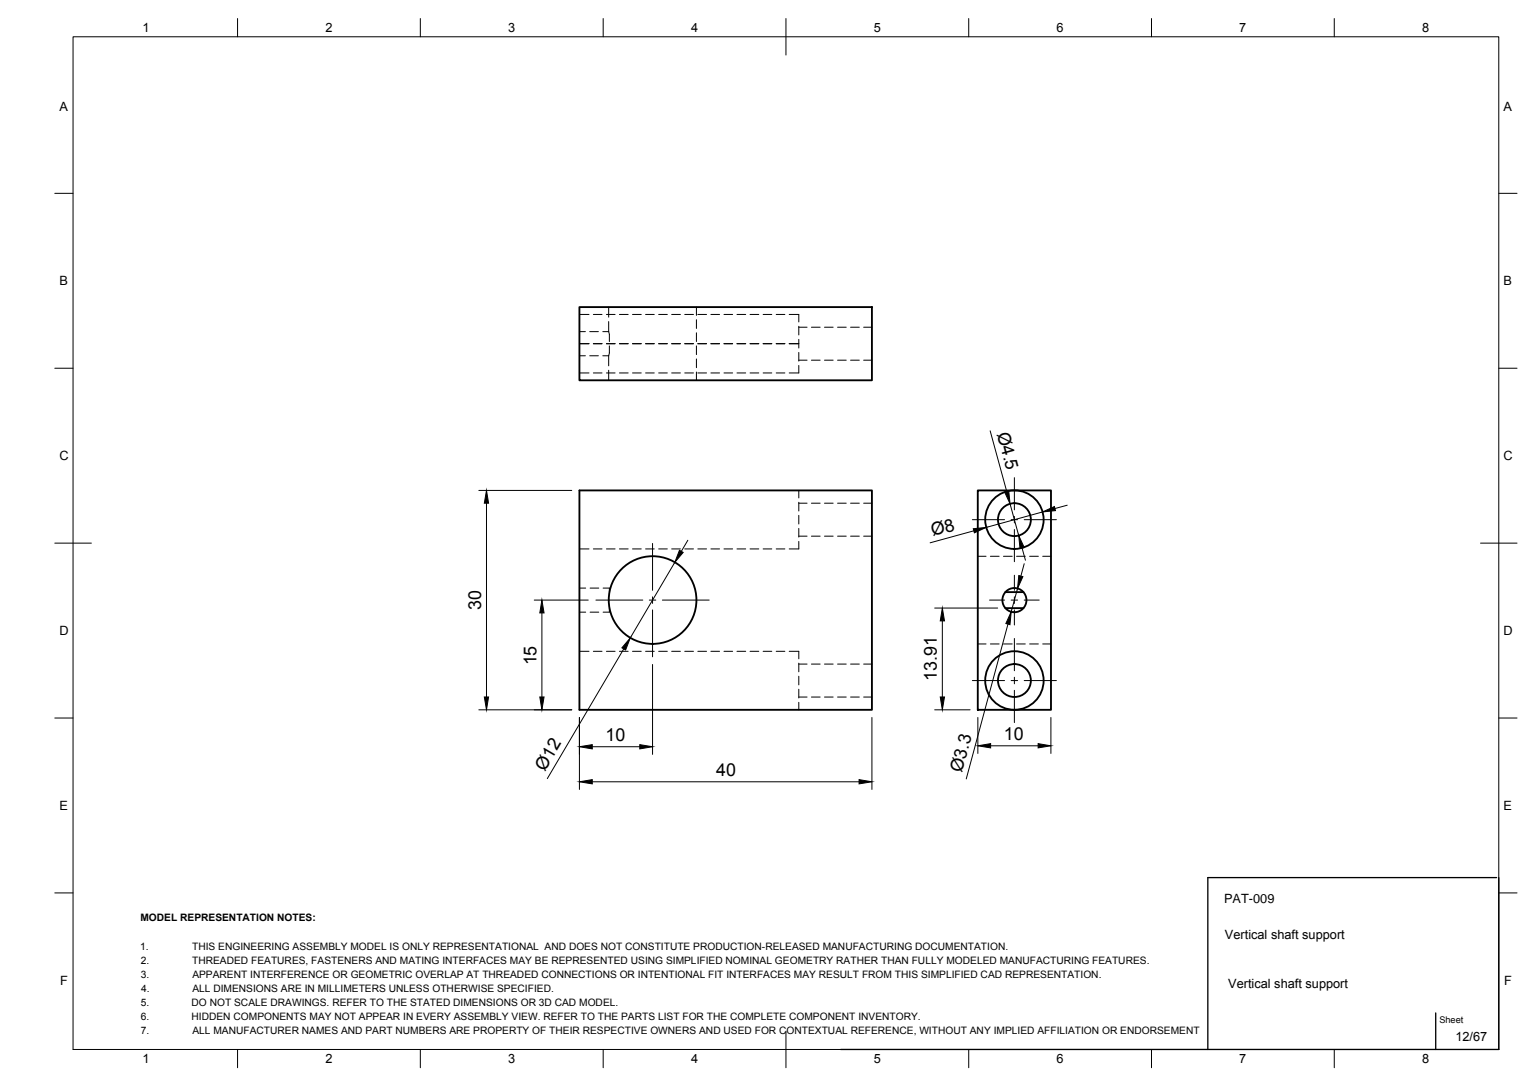
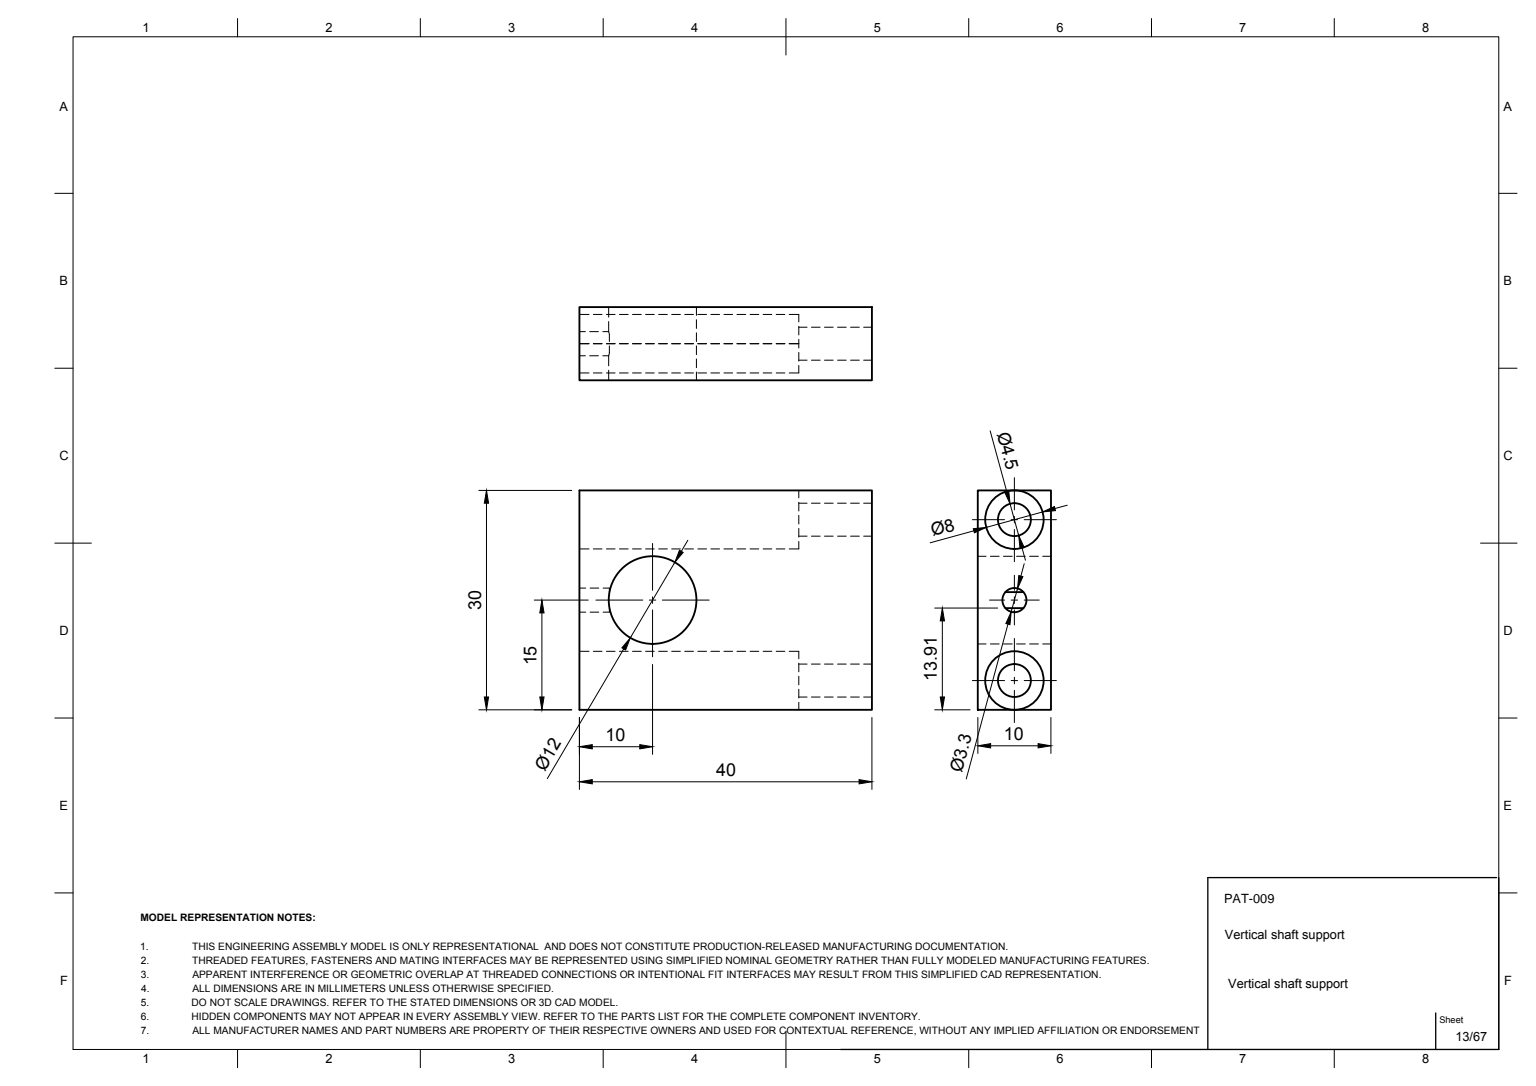
ISO-10303-21;
HEADER;
/* Generated by software containing ST-Developer
 * from STEP Tools, Inc. (www.steptools.com) 
 */

FILE_DESCRIPTION(
/* description */ ('Bell-crank linkage with push rods'),
/* implementation_level */ '2;1');

FILE_NAME(
/* name */ 'Vertical shaft support.step',
/* time_stamp */ '2026-10-28T03:25:15-07:00',
/* author */ (''),
/* organization */ (''),
/* preprocessor_version */ 'ST-DEVELOPER v20.2',
/* originating_system */ 'Autodesk Translation Framework v15.17.0.0',
/* authorisation */ '');

FILE_SCHEMA (('AUTOMOTIVE_DESIGN { 1 0 10303 214 3 1 1 }'));
ENDSEC;

DATA;
#10=MECHANICAL_DESIGN_GEOMETRIC_PRESENTATION_REPRESENTATION('',(#611),#16678);
#469=B_SPLINE_CURVE_WITH_KNOTS('',3,(#14216,#14217,#14218,#14219,#14220,
#14221,#14222,#14223,#14224,#14225),.UNSPECIFIED.,.F.,.F.,(4,2,2,2,4),(0.635430324955937,
0.687528937234029,0.750024497760675,0.81252005828732,0.864618670565412),
 .UNSPECIFIED.);
#470=B_SPLINE_CURVE_WITH_KNOTS('',3,(#14233,#14234,#14235,#14236,#14237,
#14238,#14239,#14240,#14241,#14242),.UNSPECIFIED.,.F.,.F.,(4,2,2,2,4),(0.135413993115487,
0.187512605393579,0.250008165920225,0.312503726446871,0.364602338724964),
 .UNSPECIFIED.);
#503=SHAPE_REPRESENTATION_RELATIONSHIP('SRR','None',#16919,#557);
#557=ADVANCED_BREP_SHAPE_REPRESENTATION('',(#673),#16624);
#611=STYLED_ITEM('',(#17291),#673);
#673=MANIFOLD_SOLID_BREP('Body1',#8801);
#796=FACE_BOUND('',#1959,.T.);
#797=FACE_BOUND('',#1962,.T.);
#798=FACE_BOUND('',#1964,.T.);
#799=FACE_BOUND('',#1968,.T.);
#800=FACE_BOUND('',#1970,.T.);
#801=FACE_BOUND('',#1973,.T.);
#802=FACE_BOUND('',#1976,.T.);
#803=FACE_BOUND('',#1977,.T.);
#1023=PLANE('',#9700);
#1024=PLANE('',#9706);
#1025=PLANE('',#9710);
#1026=PLANE('',#9715);
#1027=PLANE('',#9717);
#1028=PLANE('',#9725);
#1029=PLANE('',#9726);
#1030=PLANE('',#9727);
#1031=PLANE('',#9728);
#1032=PLANE('',#9729);
#1360=FACE_OUTER_BOUND('',#1953,.T.);
#1361=FACE_OUTER_BOUND('',#1954,.T.);
#1362=FACE_OUTER_BOUND('',#1955,.T.);
#1363=FACE_OUTER_BOUND('',#1956,.T.);
#1364=FACE_OUTER_BOUND('',#1957,.T.);
#1365=FACE_OUTER_BOUND('',#1958,.T.);
#1366=FACE_OUTER_BOUND('',#1960,.T.);
#1367=FACE_OUTER_BOUND('',#1961,.T.);
#1368=FACE_OUTER_BOUND('',#1963,.T.);
#1369=FACE_OUTER_BOUND('',#1965,.T.);
#1370=FACE_OUTER_BOUND('',#1966,.T.);
#1371=FACE_OUTER_BOUND('',#1967,.T.);
#1372=FACE_OUTER_BOUND('',#1969,.T.);
#1373=FACE_OUTER_BOUND('',#1971,.T.);
#1374=FACE_OUTER_BOUND('',#1972,.T.);
#1375=FACE_OUTER_BOUND('',#1974,.T.);
#1376=FACE_OUTER_BOUND('',#1975,.T.);
#1953=EDGE_LOOP('',(#6443,#6444,#6445,#6446));
#1954=EDGE_LOOP('',(#6447,#6448));
#1955=EDGE_LOOP('',(#6449,#6450,#6451,#6452,#6453,#6454,#6455,#6456));
#1956=EDGE_LOOP('',(#6457,#6458,#6459));
#1957=EDGE_LOOP('',(#6460,#6461,#6462,#6463));
#1958=EDGE_LOOP('',(#6464));
#1959=EDGE_LOOP('',(#6465));
#1960=EDGE_LOOP('',(#6466,#6467,#6468,#6469));
#1961=EDGE_LOOP('',(#6470,#6471));
#1962=EDGE_LOOP('',(#6472));
#1963=EDGE_LOOP('',(#6473,#6474,#6475,#6476,#6477,#6478,#6479,#6480,#6481));
#1964=EDGE_LOOP('',(#6482));
#1965=EDGE_LOOP('',(#6483,#6484,#6485,#6486));
#1966=EDGE_LOOP('',(#6487,#6488,#6489,#6490));
#1967=EDGE_LOOP('',(#6491,#6492,#6493,#6494));
#1968=EDGE_LOOP('',(#6495,#6496,#6497,#6498));
#1969=EDGE_LOOP('',(#6499,#6500,#6501,#6502));
#1970=EDGE_LOOP('',(#6503));
#1971=EDGE_LOOP('',(#6504,#6505,#6506,#6507,#6508,#6509,#6510));
#1972=EDGE_LOOP('',(#6511,#6512,#6513,#6514));
#1973=EDGE_LOOP('',(#6515));
#1974=EDGE_LOOP('',(#6516,#6517,#6518,#6519,#6520,#6521,#6522));
#1975=EDGE_LOOP('',(#6523,#6524,#6525,#6526));
#1976=EDGE_LOOP('',(#6527));
#1977=EDGE_LOOP('',(#6528));
#2666=LINE('',#14203,#3215);
#2667=LINE('',#14207,#3216);
#2668=LINE('',#14212,#3217);
#2669=LINE('',#14229,#3218);
#2670=LINE('',#14244,#3219);
#2671=LINE('',#14249,#3220);
#2672=LINE('',#14251,#3221);
#2673=LINE('',#14257,#3222);
#2674=LINE('',#14264,#3223);
#2675=LINE('',#14266,#3224);
#2676=LINE('',#14268,#3225);
#2677=LINE('',#14269,#3226);
#2678=LINE('',#14271,#3227);
#2679=LINE('',#14272,#3228);
#2680=LINE('',#14276,#3229);
#2681=LINE('',#14280,#3230);
#2682=LINE('',#14285,#3231);
#2683=LINE('',#14290,#3232);
#2684=LINE('',#14291,#3233);
#2685=LINE('',#14292,#3234);
#2686=LINE('',#14295,#3235);
#2687=LINE('',#14296,#3236);
#2688=LINE('',#14299,#3237);
#2689=LINE('',#14300,#3238);
#2690=LINE('',#14302,#3239);
#3215=VECTOR('',#11252,0.4);
#3216=VECTOR('',#11255,1.);
#3217=VECTOR('',#11260,1.);
#3218=VECTOR('',#11267,0.165);
#3219=VECTOR('',#11274,1.);
#3220=VECTOR('',#11279,1.);
#3221=VECTOR('',#11282,1.);
#3222=VECTOR('',#11291,1.);
#3223=VECTOR('',#11300,1.);
#3224=VECTOR('',#11301,1.);
#3225=VECTOR('',#11302,1.);
#3226=VECTOR('',#11303,1.);
#3227=VECTOR('',#11304,1.);
#3228=VECTOR('',#11305,1.);
#3229=VECTOR('',#11310,0.225);
#3230=VECTOR('',#11315,0.225);
#3231=VECTOR('',#11320,0.6);
#3232=VECTOR('',#11325,1.);
#3233=VECTOR('',#11326,1.);
#3234=VECTOR('',#11327,1.);
#3235=VECTOR('',#11330,1.);
#3236=VECTOR('',#11331,1.);
#3237=VECTOR('',#11334,1.);
#3238=VECTOR('',#11335,1.);
#3239=VECTOR('',#11338,1.);
#3750=CIRCLE('',#9698,0.4);
#3751=CIRCLE('',#9699,0.4);
#3752=CIRCLE('',#9701,0.165);
#3753=CIRCLE('',#9703,0.165);
#3754=CIRCLE('',#9704,0.165);
#3755=CIRCLE('',#9705,0.165);
#3756=CIRCLE('',#9708,0.4);
#3757=CIRCLE('',#9709,0.4);
#3758=CIRCLE('',#9711,0.225);
#3759=CIRCLE('',#9713,0.4);
#3760=CIRCLE('',#9714,0.4);
#3761=CIRCLE('',#9716,0.225);
#3762=CIRCLE('',#9719,0.225);
#3763=CIRCLE('',#9721,0.225);
#3764=CIRCLE('',#9723,0.6);
#3765=CIRCLE('',#9724,0.6);
#4292=VERTEX_POINT('',#14201);
#4293=VERTEX_POINT('',#14202);
#4294=VERTEX_POINT('',#14204);
#4295=VERTEX_POINT('',#14206);
#4296=VERTEX_POINT('',#14210);
#4297=VERTEX_POINT('',#14211);
#4298=VERTEX_POINT('',#14215);
#4299=VERTEX_POINT('',#14226);
#4300=VERTEX_POINT('',#14228);
#4301=VERTEX_POINT('',#14231);
#4302=VERTEX_POINT('',#14246);
#4303=VERTEX_POINT('',#14248);
#4304=VERTEX_POINT('',#14253);
#4305=VERTEX_POINT('',#14260);
#4306=VERTEX_POINT('',#14263);
#4307=VERTEX_POINT('',#14265);
#4308=VERTEX_POINT('',#14267);
#4309=VERTEX_POINT('',#14270);
#4310=VERTEX_POINT('',#14274);
#4311=VERTEX_POINT('',#14278);
#4312=VERTEX_POINT('',#14282);
#4313=VERTEX_POINT('',#14284);
#4314=VERTEX_POINT('',#14288);
#4315=VERTEX_POINT('',#14289);
#4316=VERTEX_POINT('',#14294);
#4317=VERTEX_POINT('',#14298);
#5099=EDGE_CURVE('',#4292,#4293,#2666,.T.);
#5100=EDGE_CURVE('',#4294,#4292,#3750,.T.);
#5101=EDGE_CURVE('',#4294,#4295,#2667,.T.);
#5102=EDGE_CURVE('',#4293,#4295,#3751,.T.);
#5103=EDGE_CURVE('',#4296,#4297,#2668,.T.);
#5104=EDGE_CURVE('',#4296,#4297,#3752,.T.);
#5105=EDGE_CURVE('',#4298,#4296,#469,.T.);
#5106=EDGE_CURVE('',#4299,#4298,#3753,.T.);
#5107=EDGE_CURVE('',#4299,#4300,#2669,.T.);
#5108=EDGE_CURVE('',#4300,#4300,#3754,.T.);
#5109=EDGE_CURVE('',#4301,#4299,#3755,.T.);
#5110=EDGE_CURVE('',#4297,#4301,#470,.T.);
#5111=EDGE_CURVE('',#4301,#4298,#2670,.T.);
#5112=EDGE_CURVE('',#4302,#4302,#3756,.T.);
#5113=EDGE_CURVE('',#4302,#4303,#2671,.T.);
#5114=EDGE_CURVE('',#4303,#4303,#3757,.T.);
#5115=EDGE_CURVE('',#4302,#4303,#2672,.T.);
#5116=EDGE_CURVE('',#4304,#4304,#3758,.T.);
#5117=EDGE_CURVE('',#4295,#4293,#3759,.T.);
#5118=EDGE_CURVE('',#4294,#4295,#2673,.T.);
#5119=EDGE_CURVE('',#4292,#4294,#3760,.T.);
#5120=EDGE_CURVE('',#4305,#4305,#3761,.T.);
#5121=EDGE_CURVE('',#4306,#4303,#2674,.T.);
#5122=EDGE_CURVE('',#4303,#4307,#2675,.T.);
#5123=EDGE_CURVE('',#4307,#4308,#2676,.T.);
#5124=EDGE_CURVE('',#4308,#4295,#2677,.T.);
#5125=EDGE_CURVE('',#4295,#4309,#2678,.T.);
#5126=EDGE_CURVE('',#4309,#4306,#2679,.T.);
#5127=EDGE_CURVE('',#4310,#4310,#3762,.T.);
#5128=EDGE_CURVE('',#4310,#4304,#2680,.T.);
#5129=EDGE_CURVE('',#4311,#4311,#3763,.T.);
#5130=EDGE_CURVE('',#4311,#4305,#2681,.T.);
#5131=EDGE_CURVE('',#4312,#4312,#3764,.T.);
#5132=EDGE_CURVE('',#4312,#4313,#2682,.T.);
#5133=EDGE_CURVE('',#4313,#4313,#3765,.T.);
#5134=EDGE_CURVE('',#4314,#4315,#2683,.T.);
#5135=EDGE_CURVE('',#4315,#4306,#2684,.T.);
#5136=EDGE_CURVE('',#4314,#4309,#2685,.T.);
#5137=EDGE_CURVE('',#4316,#4314,#2686,.T.);
#5138=EDGE_CURVE('',#4316,#4308,#2687,.T.);
#5139=EDGE_CURVE('',#4317,#4316,#2688,.T.);
#5140=EDGE_CURVE('',#4317,#4307,#2689,.T.);
#5141=EDGE_CURVE('',#4315,#4317,#2690,.T.);
#6443=ORIENTED_EDGE('',*,*,#5099,.F.);
#6444=ORIENTED_EDGE('',*,*,#5100,.F.);
#6445=ORIENTED_EDGE('',*,*,#5101,.T.);
#6446=ORIENTED_EDGE('',*,*,#5102,.F.);
#6447=ORIENTED_EDGE('',*,*,#5103,.F.);
#6448=ORIENTED_EDGE('',*,*,#5104,.T.);
#6449=ORIENTED_EDGE('',*,*,#5105,.F.);
#6450=ORIENTED_EDGE('',*,*,#5106,.F.);
#6451=ORIENTED_EDGE('',*,*,#5107,.T.);
#6452=ORIENTED_EDGE('',*,*,#5108,.F.);
#6453=ORIENTED_EDGE('',*,*,#5107,.F.);
#6454=ORIENTED_EDGE('',*,*,#5109,.F.);
#6455=ORIENTED_EDGE('',*,*,#5110,.F.);
#6456=ORIENTED_EDGE('',*,*,#5104,.F.);
#6457=ORIENTED_EDGE('',*,*,#5111,.F.);
#6458=ORIENTED_EDGE('',*,*,#5109,.T.);
#6459=ORIENTED_EDGE('',*,*,#5106,.T.);
#6460=ORIENTED_EDGE('',*,*,#5112,.F.);
#6461=ORIENTED_EDGE('',*,*,#5113,.T.);
#6462=ORIENTED_EDGE('',*,*,#5114,.F.);
#6463=ORIENTED_EDGE('',*,*,#5115,.F.);
#6464=ORIENTED_EDGE('',*,*,#5112,.T.);
#6465=ORIENTED_EDGE('',*,*,#5116,.F.);
#6466=ORIENTED_EDGE('',*,*,#5099,.T.);
#6467=ORIENTED_EDGE('',*,*,#5117,.F.);
#6468=ORIENTED_EDGE('',*,*,#5118,.F.);
#6469=ORIENTED_EDGE('',*,*,#5119,.F.);
#6470=ORIENTED_EDGE('',*,*,#5100,.T.);
#6471=ORIENTED_EDGE('',*,*,#5119,.T.);
#6472=ORIENTED_EDGE('',*,*,#5120,.F.);
#6473=ORIENTED_EDGE('',*,*,#5121,.T.);
#6474=ORIENTED_EDGE('',*,*,#5114,.T.);
#6475=ORIENTED_EDGE('',*,*,#5122,.T.);
#6476=ORIENTED_EDGE('',*,*,#5123,.T.);
#6477=ORIENTED_EDGE('',*,*,#5124,.T.);
#6478=ORIENTED_EDGE('',*,*,#5117,.T.);
#6479=ORIENTED_EDGE('',*,*,#5102,.T.);
#6480=ORIENTED_EDGE('',*,*,#5125,.T.);
#6481=ORIENTED_EDGE('',*,*,#5126,.T.);
#6482=ORIENTED_EDGE('',*,*,#5108,.T.);
#6483=ORIENTED_EDGE('',*,*,#5127,.F.);
#6484=ORIENTED_EDGE('',*,*,#5128,.T.);
#6485=ORIENTED_EDGE('',*,*,#5116,.T.);
#6486=ORIENTED_EDGE('',*,*,#5128,.F.);
#6487=ORIENTED_EDGE('',*,*,#5129,.F.);
#6488=ORIENTED_EDGE('',*,*,#5130,.T.);
#6489=ORIENTED_EDGE('',*,*,#5120,.T.);
#6490=ORIENTED_EDGE('',*,*,#5130,.F.);
#6491=ORIENTED_EDGE('',*,*,#5131,.F.);
#6492=ORIENTED_EDGE('',*,*,#5132,.T.);
#6493=ORIENTED_EDGE('',*,*,#5133,.F.);
#6494=ORIENTED_EDGE('',*,*,#5132,.F.);
#6495=ORIENTED_EDGE('',*,*,#5110,.T.);
#6496=ORIENTED_EDGE('',*,*,#5111,.T.);
#6497=ORIENTED_EDGE('',*,*,#5105,.T.);
#6498=ORIENTED_EDGE('',*,*,#5103,.T.);
#6499=ORIENTED_EDGE('',*,*,#5134,.T.);
#6500=ORIENTED_EDGE('',*,*,#5135,.T.);
#6501=ORIENTED_EDGE('',*,*,#5126,.F.);
#6502=ORIENTED_EDGE('',*,*,#5136,.F.);
#6503=ORIENTED_EDGE('',*,*,#5133,.T.);
#6504=ORIENTED_EDGE('',*,*,#5137,.T.);
#6505=ORIENTED_EDGE('',*,*,#5136,.T.);
#6506=ORIENTED_EDGE('',*,*,#5125,.F.);
#6507=ORIENTED_EDGE('',*,*,#5101,.F.);
#6508=ORIENTED_EDGE('',*,*,#5118,.T.);
#6509=ORIENTED_EDGE('',*,*,#5124,.F.);
#6510=ORIENTED_EDGE('',*,*,#5138,.F.);
#6511=ORIENTED_EDGE('',*,*,#5139,.T.);
#6512=ORIENTED_EDGE('',*,*,#5138,.T.);
#6513=ORIENTED_EDGE('',*,*,#5123,.F.);
#6514=ORIENTED_EDGE('',*,*,#5140,.F.);
#6515=ORIENTED_EDGE('',*,*,#5131,.T.);
#6516=ORIENTED_EDGE('',*,*,#5141,.T.);
#6517=ORIENTED_EDGE('',*,*,#5140,.T.);
#6518=ORIENTED_EDGE('',*,*,#5122,.F.);
#6519=ORIENTED_EDGE('',*,*,#5113,.F.);
#6520=ORIENTED_EDGE('',*,*,#5115,.T.);
#6521=ORIENTED_EDGE('',*,*,#5121,.F.);
#6522=ORIENTED_EDGE('',*,*,#5135,.F.);
#6523=ORIENTED_EDGE('',*,*,#5141,.F.);
#6524=ORIENTED_EDGE('',*,*,#5134,.F.);
#6525=ORIENTED_EDGE('',*,*,#5137,.F.);
#6526=ORIENTED_EDGE('',*,*,#5139,.F.);
#6527=ORIENTED_EDGE('',*,*,#5127,.T.);
#6528=ORIENTED_EDGE('',*,*,#5129,.T.);
#8123=CYLINDRICAL_SURFACE('',#9697,0.4);
#8124=CYLINDRICAL_SURFACE('',#9702,0.165);
#8125=CYLINDRICAL_SURFACE('',#9707,0.4);
#8126=CYLINDRICAL_SURFACE('',#9712,0.4);
#8127=CYLINDRICAL_SURFACE('',#9718,0.225);
#8128=CYLINDRICAL_SURFACE('',#9720,0.225);
#8129=CYLINDRICAL_SURFACE('',#9722,0.6);
#8385=ADVANCED_FACE('',(#1360),#8123,.F.);
#8386=ADVANCED_FACE('',(#1361),#1023,.T.);
#8387=ADVANCED_FACE('',(#1362),#8124,.F.);
#8388=ADVANCED_FACE('',(#1363),#1024,.T.);
#8389=ADVANCED_FACE('',(#1364),#8125,.F.);
#8390=ADVANCED_FACE('',(#1365,#796),#1025,.T.);
#8391=ADVANCED_FACE('',(#1366),#8126,.F.);
#8392=ADVANCED_FACE('',(#1367,#797),#1026,.T.);
#8393=ADVANCED_FACE('',(#1368,#798),#1027,.T.);
#8394=ADVANCED_FACE('',(#1369),#8127,.F.);
#8395=ADVANCED_FACE('',(#1370),#8128,.F.);
#8396=ADVANCED_FACE('',(#1371,#799),#8129,.F.);
#8397=ADVANCED_FACE('',(#1372,#800),#1028,.T.);
#8398=ADVANCED_FACE('',(#1373),#1029,.T.);
#8399=ADVANCED_FACE('',(#1374,#801),#1030,.T.);
#8400=ADVANCED_FACE('',(#1375),#1031,.T.);
#8401=ADVANCED_FACE('',(#1376,#802,#803),#1032,.F.);
#8801=CLOSED_SHELL('',(#8385,#8386,#8387,#8388,#8389,#8390,#8391,#8392,
#8393,#8394,#8395,#8396,#8397,#8398,#8399,#8400,#8401));
#9696=AXIS2_PLACEMENT_3D('',#14199,#11248,#11249);
#9697=AXIS2_PLACEMENT_3D('',#14200,#11250,#11251);
#9698=AXIS2_PLACEMENT_3D('',#14205,#11253,#11254);
#9699=AXIS2_PLACEMENT_3D('',#14208,#11256,#11257);
#9700=AXIS2_PLACEMENT_3D('',#14209,#11258,#11259);
#9701=AXIS2_PLACEMENT_3D('',#14213,#11261,#11262);
#9702=AXIS2_PLACEMENT_3D('',#14214,#11263,#11264);
#9703=AXIS2_PLACEMENT_3D('',#14227,#11265,#11266);
#9704=AXIS2_PLACEMENT_3D('',#14230,#11268,#11269);
#9705=AXIS2_PLACEMENT_3D('',#14232,#11270,#11271);
#9706=AXIS2_PLACEMENT_3D('',#14243,#11272,#11273);
#9707=AXIS2_PLACEMENT_3D('',#14245,#11275,#11276);
#9708=AXIS2_PLACEMENT_3D('',#14247,#11277,#11278);
#9709=AXIS2_PLACEMENT_3D('',#14250,#11280,#11281);
#9710=AXIS2_PLACEMENT_3D('',#14252,#11283,#11284);
#9711=AXIS2_PLACEMENT_3D('',#14254,#11285,#11286);
#9712=AXIS2_PLACEMENT_3D('',#14255,#11287,#11288);
#9713=AXIS2_PLACEMENT_3D('',#14256,#11289,#11290);
#9714=AXIS2_PLACEMENT_3D('',#14258,#11292,#11293);
#9715=AXIS2_PLACEMENT_3D('',#14259,#11294,#11295);
#9716=AXIS2_PLACEMENT_3D('',#14261,#11296,#11297);
#9717=AXIS2_PLACEMENT_3D('',#14262,#11298,#11299);
#9718=AXIS2_PLACEMENT_3D('',#14273,#11306,#11307);
#9719=AXIS2_PLACEMENT_3D('',#14275,#11308,#11309);
#9720=AXIS2_PLACEMENT_3D('',#14277,#11311,#11312);
#9721=AXIS2_PLACEMENT_3D('',#14279,#11313,#11314);
#9722=AXIS2_PLACEMENT_3D('',#14281,#11316,#11317);
#9723=AXIS2_PLACEMENT_3D('',#14283,#11318,#11319);
#9724=AXIS2_PLACEMENT_3D('',#14286,#11321,#11322);
#9725=AXIS2_PLACEMENT_3D('',#14287,#11323,#11324);
#9726=AXIS2_PLACEMENT_3D('',#14293,#11328,#11329);
#9727=AXIS2_PLACEMENT_3D('',#14297,#11332,#11333);
#9728=AXIS2_PLACEMENT_3D('',#14301,#11336,#11337);
#9729=AXIS2_PLACEMENT_3D('',#14303,#11339,#11340);
#11248=DIRECTION('axis',(0.,0.,1.));
#11249=DIRECTION('refdir',(1.,0.,0.));
#11250=DIRECTION('center_axis',(0.,0.,1.));
#11251=DIRECTION('ref_axis',(1.,0.,0.));
#11252=DIRECTION('',(0.,0.,1.));
#11253=DIRECTION('center_axis',(0.,0.,1.));
#11254=DIRECTION('ref_axis',(1.,0.,0.));
#11255=DIRECTION('',(0.,0.,1.));
#11256=DIRECTION('center_axis',(0.,0.,-1.));
#11257=DIRECTION('ref_axis',(1.,0.,0.));
#11258=DIRECTION('center_axis',(0.,0.,1.));
#11259=DIRECTION('ref_axis',(1.,0.,0.));
#11260=DIRECTION('',(0.,1.,0.));
#11261=DIRECTION('center_axis',(0.,0.,1.));
#11262=DIRECTION('ref_axis',(1.,0.,0.));
#11263=DIRECTION('center_axis',(0.,0.,1.));
#11264=DIRECTION('ref_axis',(1.,0.,0.));
#11265=DIRECTION('center_axis',(0.,0.,1.));
#11266=DIRECTION('ref_axis',(1.,0.,0.));
#11267=DIRECTION('',(0.,0.,1.));
#11268=DIRECTION('center_axis',(0.,0.,-1.));
#11269=DIRECTION('ref_axis',(1.,0.,0.));
#11270=DIRECTION('center_axis',(0.,0.,1.));
#11271=DIRECTION('ref_axis',(1.,0.,0.));
#11272=DIRECTION('center_axis',(0.,0.,1.));
#11273=DIRECTION('ref_axis',(1.,0.,0.));
#11274=DIRECTION('',(0.,-1.,0.));
#11275=DIRECTION('center_axis',(0.,0.,1.));
#11276=DIRECTION('ref_axis',(1.,0.,0.));
#11277=DIRECTION('center_axis',(0.,0.,1.));
#11278=DIRECTION('ref_axis',(1.,0.,0.));
#11279=DIRECTION('',(0.,0.,1.));
#11280=DIRECTION('center_axis',(0.,0.,-1.));
#11281=DIRECTION('ref_axis',(1.,0.,0.));
#11282=DIRECTION('',(0.,0.,1.));
#11283=DIRECTION('center_axis',(0.,0.,1.));
#11284=DIRECTION('ref_axis',(1.,0.,0.));
#11285=DIRECTION('center_axis',(0.,0.,1.));
#11286=DIRECTION('ref_axis',(1.,0.,0.));
#11287=DIRECTION('center_axis',(0.,0.,1.));
#11288=DIRECTION('ref_axis',(1.,0.,0.));
#11289=DIRECTION('center_axis',(0.,0.,-1.));
#11290=DIRECTION('ref_axis',(1.,0.,0.));
#11291=DIRECTION('',(0.,0.,1.));
#11292=DIRECTION('center_axis',(0.,0.,1.));
#11293=DIRECTION('ref_axis',(1.,0.,0.));
#11294=DIRECTION('center_axis',(0.,0.,1.));
#11295=DIRECTION('ref_axis',(1.,0.,0.));
#11296=DIRECTION('center_axis',(0.,0.,1.));
#11297=DIRECTION('ref_axis',(1.,0.,0.));
#11298=DIRECTION('center_axis',(0.,0.,1.));
#11299=DIRECTION('ref_axis',(1.,0.,0.));
#11300=DIRECTION('',(0.,-1.,0.));
#11301=DIRECTION('',(0.,-1.,0.));
#11302=DIRECTION('',(1.,0.,0.));
#11303=DIRECTION('',(0.,1.,0.));
#11304=DIRECTION('',(0.,1.,0.));
#11305=DIRECTION('',(-1.,0.,0.));
#11306=DIRECTION('center_axis',(0.,0.,1.));
#11307=DIRECTION('ref_axis',(1.,0.,0.));
#11308=DIRECTION('center_axis',(0.,0.,1.));
#11309=DIRECTION('ref_axis',(1.,0.,0.));
#11310=DIRECTION('',(0.,0.,1.));
#11311=DIRECTION('center_axis',(0.,0.,1.));
#11312=DIRECTION('ref_axis',(1.,0.,0.));
#11313=DIRECTION('center_axis',(0.,0.,1.));
#11314=DIRECTION('ref_axis',(1.,0.,0.));
#11315=DIRECTION('',(0.,0.,1.));
#11316=DIRECTION('center_axis',(0.,1.,0.));
#11317=DIRECTION('ref_axis',(1.,0.,0.));
#11318=DIRECTION('center_axis',(0.,1.,0.));
#11319=DIRECTION('ref_axis',(1.,0.,0.));
#11320=DIRECTION('',(0.,1.,0.));
#11321=DIRECTION('center_axis',(0.,-1.,0.));
#11322=DIRECTION('ref_axis',(1.,0.,0.));
#11323=DIRECTION('center_axis',(0.,1.,0.));
#11324=DIRECTION('ref_axis',(-1.,0.,0.));
#11325=DIRECTION('',(-1.,0.,0.));
#11326=DIRECTION('',(0.,0.,1.));
#11327=DIRECTION('',(0.,0.,1.));
#11328=DIRECTION('center_axis',(1.,0.,0.));
#11329=DIRECTION('ref_axis',(0.,1.,0.));
#11330=DIRECTION('',(0.,1.,0.));
#11331=DIRECTION('',(0.,0.,1.));
#11332=DIRECTION('center_axis',(0.,-1.,0.));
#11333=DIRECTION('ref_axis',(1.,0.,0.));
#11334=DIRECTION('',(1.,0.,0.));
#11335=DIRECTION('',(0.,0.,1.));
#11336=DIRECTION('center_axis',(-1.,0.,0.));
#11337=DIRECTION('ref_axis',(0.,-1.,0.));
#11338=DIRECTION('',(0.,-1.,0.));
#11339=DIRECTION('center_axis',(0.,0.,1.));
#11340=DIRECTION('ref_axis',(1.,0.,0.));
#14199=CARTESIAN_POINT('',(0.,0.,0.));
#14200=CARTESIAN_POINT('Origin',(5.1,7.5,2.));
#14201=CARTESIAN_POINT('',(4.7,7.5,2.));
#14202=CARTESIAN_POINT('',(4.7,7.5,5.));
#14203=CARTESIAN_POINT('',(4.7,7.5,2.));
#14204=CARTESIAN_POINT('',(5.5,7.5,2.));
#14205=CARTESIAN_POINT('Origin',(5.1,7.5,2.));
#14206=CARTESIAN_POINT('',(5.5,7.5,5.));
#14207=CARTESIAN_POINT('',(5.5,7.5,2.));
#14208=CARTESIAN_POINT('Origin',(5.1,7.5,5.));
#14209=CARTESIAN_POINT('Origin',(4.,7.5,4.59));
#14210=CARTESIAN_POINT('',(4.10908712114636,7.3762058159686,4.59));
#14211=CARTESIAN_POINT('',(4.10908712114636,7.6237941840314,4.59));
#14212=CARTESIAN_POINT('',(4.10908712114636,6.9,4.59));
#14213=CARTESIAN_POINT('Origin',(4.,7.5,4.59));
#14214=CARTESIAN_POINT('Origin',(4.,7.5,4.59));
#14215=CARTESIAN_POINT('',(3.89091287885364,7.3762058159686,4.59));
#14216=CARTESIAN_POINT('Ctrl Pts',(3.89091287885364,7.3762058159686,4.59));
#14217=CARTESIAN_POINT('Ctrl Pts',(3.90408240284739,7.36460086481046,4.59243495840567));
#14218=CARTESIAN_POINT('Ctrl Pts',(3.91977655056228,7.35465435634175,4.59485638705045));
#14219=CARTESIAN_POINT('Ctrl Pts',(3.95701983403981,7.33918513536598,4.59880705606552));
#14220=CARTESIAN_POINT('Ctrl Pts',(3.97916814649112,7.335,4.6));
#14221=CARTESIAN_POINT('Ctrl Pts',(4.02083185350888,7.335,4.6));
#14222=CARTESIAN_POINT('Ctrl Pts',(4.04298016596019,7.33918513536598,4.59880705606552));
#14223=CARTESIAN_POINT('Ctrl Pts',(4.08022344943772,7.35465435634175,4.59485638705045));
#14224=CARTESIAN_POINT('Ctrl Pts',(4.09591759715261,7.36460086481046,4.59243495840567));
#14225=CARTESIAN_POINT('Ctrl Pts',(4.10908712114636,7.3762058159686,4.59));
#14226=CARTESIAN_POINT('',(3.835,7.5,4.59));
#14227=CARTESIAN_POINT('Origin',(4.,7.5,4.59));
#14228=CARTESIAN_POINT('',(3.835,7.5,5.));
#14229=CARTESIAN_POINT('',(3.835,7.5,4.59));
#14230=CARTESIAN_POINT('Origin',(4.,7.5,5.));
#14231=CARTESIAN_POINT('',(3.89091287885364,7.6237941840314,4.59));
#14232=CARTESIAN_POINT('Origin',(4.,7.5,4.59));
#14233=CARTESIAN_POINT('Ctrl Pts',(4.10908712114636,7.6237941840314,4.59));
#14234=CARTESIAN_POINT('Ctrl Pts',(4.09591759715261,7.63539913518953,4.59243495840567));
#14235=CARTESIAN_POINT('Ctrl Pts',(4.08022344943772,7.64534564365825,4.59485638705045));
#14236=CARTESIAN_POINT('Ctrl Pts',(4.04298016596019,7.66081486463402,4.59880705606552));
#14237=CARTESIAN_POINT('Ctrl Pts',(4.02083185350888,7.665,4.6));
#14238=CARTESIAN_POINT('Ctrl Pts',(3.97916814649112,7.665,4.6));
#14239=CARTESIAN_POINT('Ctrl Pts',(3.95701983403981,7.66081486463402,4.59880705606552));
#14240=CARTESIAN_POINT('Ctrl Pts',(3.91977655056228,7.64534564365825,4.59485638705045));
#14241=CARTESIAN_POINT('Ctrl Pts',(3.90408240284739,7.63539913518954,4.59243495840567));
#14242=CARTESIAN_POINT('Ctrl Pts',(3.89091287885364,7.6237941840314,4.59));
#14243=CARTESIAN_POINT('Origin',(4.,7.5,4.59));
#14244=CARTESIAN_POINT('',(3.89091287885364,6.9,4.59));
#14245=CARTESIAN_POINT('Origin',(2.9,7.5,2.));
#14246=CARTESIAN_POINT('',(2.5,7.5,2.));
#14247=CARTESIAN_POINT('Origin',(2.9,7.5,2.));
#14248=CARTESIAN_POINT('',(2.5,7.5,5.));
#14249=CARTESIAN_POINT('',(2.5,7.5,2.));
#14250=CARTESIAN_POINT('Origin',(2.9,7.5,5.));
#14251=CARTESIAN_POINT('',(2.5,7.5,2.));
#14252=CARTESIAN_POINT('Origin',(2.9,7.5,2.));
#14253=CARTESIAN_POINT('',(2.675,7.5,2.));
#14254=CARTESIAN_POINT('Origin',(2.9,7.5,2.));
#14255=CARTESIAN_POINT('Origin',(5.1,7.5,2.));
#14256=CARTESIAN_POINT('Origin',(5.1,7.5,5.));
#14257=CARTESIAN_POINT('',(5.5,7.5,2.));
#14258=CARTESIAN_POINT('Origin',(5.1,7.5,2.));
#14259=CARTESIAN_POINT('Origin',(5.1,7.5,2.));
#14260=CARTESIAN_POINT('',(4.875,7.5,2.));
#14261=CARTESIAN_POINT('Origin',(5.1,7.5,2.));
#14262=CARTESIAN_POINT('Origin',(4.,7.5,5.));
#14263=CARTESIAN_POINT('',(2.5,8.,5.));
#14264=CARTESIAN_POINT('',(2.5,8.,5.));
#14265=CARTESIAN_POINT('',(2.5,7.,5.));
#14266=CARTESIAN_POINT('',(2.5,8.,5.));
#14267=CARTESIAN_POINT('',(5.5,7.,5.));
#14268=CARTESIAN_POINT('',(2.5,7.,5.));
#14269=CARTESIAN_POINT('',(5.5,7.,5.));
#14270=CARTESIAN_POINT('',(5.5,8.,5.));
#14271=CARTESIAN_POINT('',(5.5,7.,5.));
#14272=CARTESIAN_POINT('',(5.5,8.,5.));
#14273=CARTESIAN_POINT('Origin',(2.9,7.5,0.9));
#14274=CARTESIAN_POINT('',(2.675,7.5,1.));
#14275=CARTESIAN_POINT('Origin',(2.9,7.5,1.));
#14276=CARTESIAN_POINT('',(2.675,7.5,0.9));
#14277=CARTESIAN_POINT('Origin',(5.1,7.5,0.9));
#14278=CARTESIAN_POINT('',(4.875,7.5,1.));
#14279=CARTESIAN_POINT('Origin',(5.1,7.5,1.));
#14280=CARTESIAN_POINT('',(4.875,7.5,0.9));
#14281=CARTESIAN_POINT('Origin',(4.,6.9,4.));
#14282=CARTESIAN_POINT('',(3.4,7.,4.));
#14283=CARTESIAN_POINT('Origin',(4.,7.,4.));
#14284=CARTESIAN_POINT('',(3.4,8.,4.));
#14285=CARTESIAN_POINT('',(3.4,6.9,4.));
#14286=CARTESIAN_POINT('Origin',(4.,8.,4.));
#14287=CARTESIAN_POINT('Origin',(5.5,8.,1.));
#14288=CARTESIAN_POINT('',(5.5,8.,1.));
#14289=CARTESIAN_POINT('',(2.5,8.,1.));
#14290=CARTESIAN_POINT('',(5.5,8.,1.));
#14291=CARTESIAN_POINT('',(2.5,8.,1.));
#14292=CARTESIAN_POINT('',(5.5,8.,1.));
#14293=CARTESIAN_POINT('Origin',(5.5,7.,1.));
#14294=CARTESIAN_POINT('',(5.5,7.,1.));
#14295=CARTESIAN_POINT('',(5.5,7.,1.));
#14296=CARTESIAN_POINT('',(5.5,7.,1.));
#14297=CARTESIAN_POINT('Origin',(2.5,7.,1.));
#14298=CARTESIAN_POINT('',(2.5,7.,1.));
#14299=CARTESIAN_POINT('',(2.5,7.,1.));
#14300=CARTESIAN_POINT('',(2.5,7.,1.));
#14301=CARTESIAN_POINT('Origin',(2.5,8.,1.));
#14302=CARTESIAN_POINT('',(2.5,8.,1.));
#14303=CARTESIAN_POINT('Origin',(4.,7.5,1.));
#16560=UNCERTAINTY_MEASURE_WITH_UNIT(LENGTH_MEASURE(0.001),#16679,
'DISTANCE_ACCURACY_VALUE',
'Maximum model space distance between geometric entities at asserted c
onnectivities');
#16614=UNCERTAINTY_MEASURE_WITH_UNIT(LENGTH_MEASURE(0.001),#16679,
'DISTANCE_ACCURACY_VALUE',
'Maximum model space distance between geometric entities at asserted c
onnectivities');
#16624=(
GEOMETRIC_REPRESENTATION_CONTEXT(3)
GLOBAL_UNCERTAINTY_ASSIGNED_CONTEXT((#16560))
GLOBAL_UNIT_ASSIGNED_CONTEXT((#16679,#16681,#16682))
REPRESENTATION_CONTEXT('','3D')
);
#16678=(
GEOMETRIC_REPRESENTATION_CONTEXT(3)
GLOBAL_UNCERTAINTY_ASSIGNED_CONTEXT((#16614))
GLOBAL_UNIT_ASSIGNED_CONTEXT((#16679,#16681,#16682))
REPRESENTATION_CONTEXT('','3D')
);
#16679=(
LENGTH_UNIT()
NAMED_UNIT(*)
SI_UNIT(.CENTI.,.METRE.)
);
#16681=(
NAMED_UNIT(*)
PLANE_ANGLE_UNIT()
SI_UNIT($,.RADIAN.)
);
#16682=(
NAMED_UNIT(*)
SI_UNIT($,.STERADIAN.)
SOLID_ANGLE_UNIT()
);
#16692=SHAPE_DEFINITION_REPRESENTATION(#16755,#16919);
#16755=PRODUCT_DEFINITION_SHAPE('',$,#16983);
#16919=SHAPE_REPRESENTATION('',(#9696),#16624);
#16973=PRODUCT_DEFINITION_CONTEXT('part definition',#17164,'design');
#16983=PRODUCT_DEFINITION('Vertical shaft support',
'Vertical shaft support',#17046,#16973);
#17046=PRODUCT_DEFINITION_FORMATION('',$,#17175);
#17164=APPLICATION_CONTEXT(
'Core Data for Automotive Mechanical Design Process');
#17165=PRODUCT_CONTEXT('part definition',#17164,'mechanical');
#17175=PRODUCT('Vertical shaft support','Vertical shaft support',
'Vertical shaft support',(#17165));
#17285=COLOUR_RGB('Grey',0.48,0.52,0.57);
#17286=FILL_AREA_STYLE_COLOUR('',#17285);
#17287=FILL_AREA_STYLE('',(#17286));
#17288=SURFACE_STYLE_FILL_AREA(#17287);
#17289=SURFACE_SIDE_STYLE('',(#17288));
#17290=SURFACE_STYLE_USAGE(.BOTH.,#17289);
#17291=PRESENTATION_STYLE_ASSIGNMENT((#17290));
ENDSEC;
END-ISO-10303-21;
